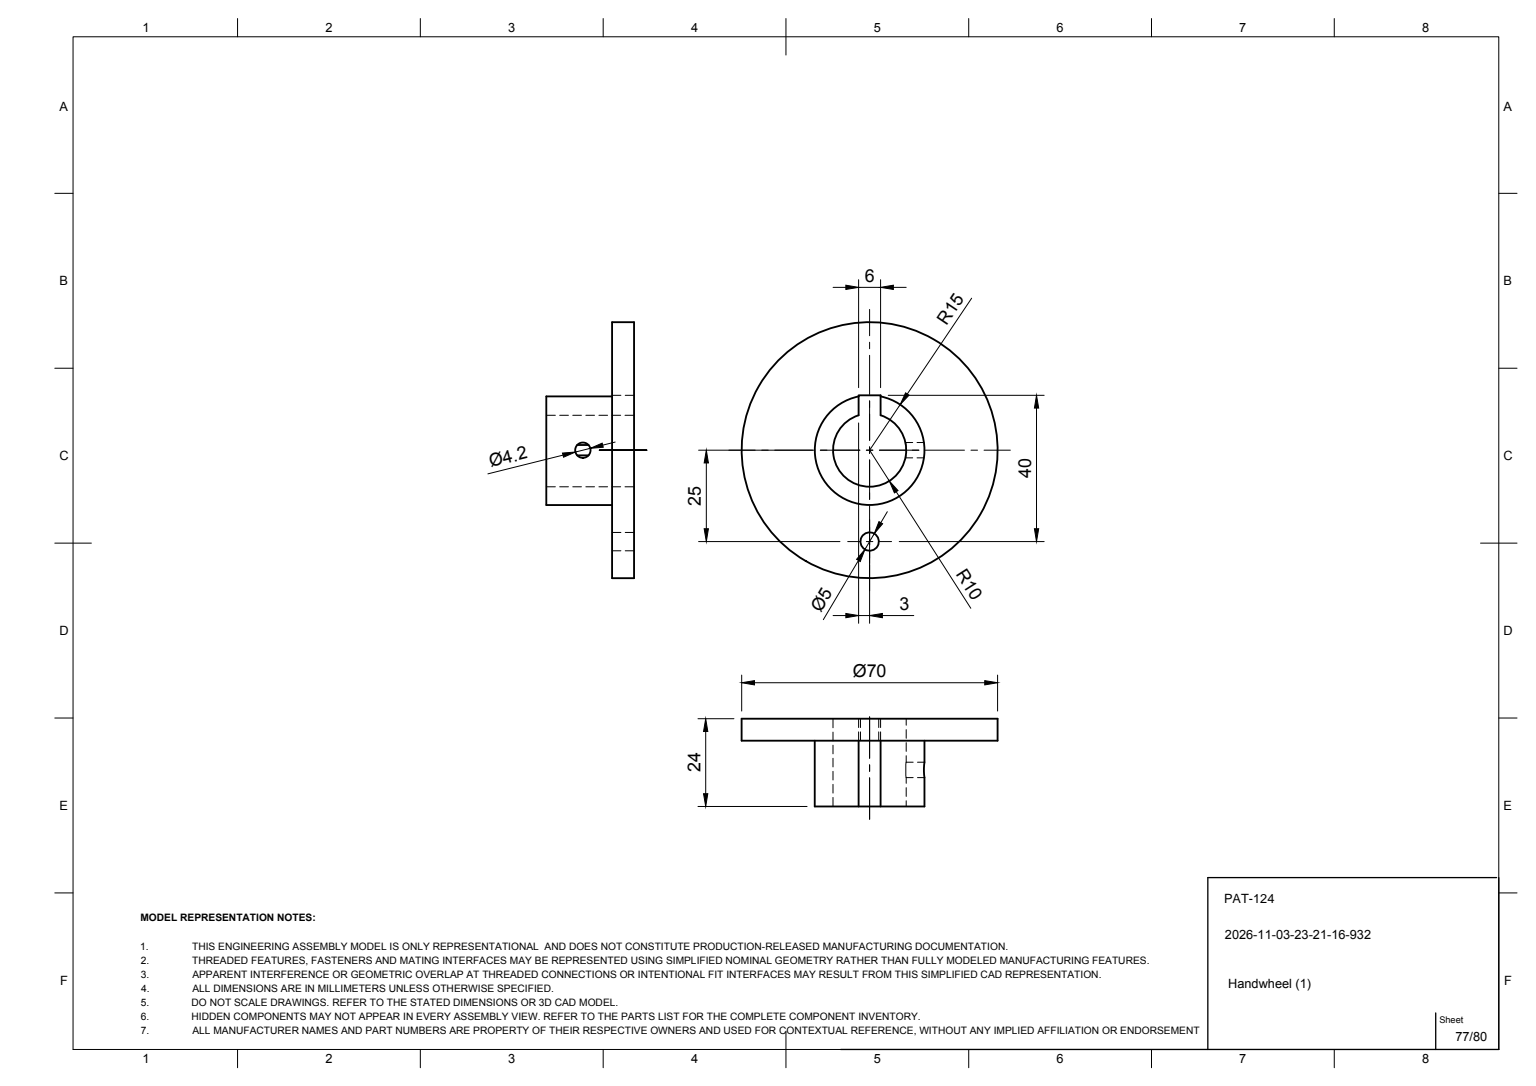
ISO-10303-21;
HEADER;
/* Generated by software containing ST-Developer
 * from STEP Tools, Inc. (www.steptools.com) 
 */

FILE_DESCRIPTION(
/* description */ ('XY cross-slide table'),
/* implementation_level */ '2;1');

FILE_NAME(
/* name */ 'Handwheel (1).step',
/* time_stamp */ '2026-10-28T03:22:46-07:00',
/* author */ (''),
/* organization */ (''),
/* preprocessor_version */ 'ST-DEVELOPER v20.2',
/* originating_system */ 'Autodesk Translation Framework v15.17.0.0',
/* authorisation */ '');

FILE_SCHEMA (('AUTOMOTIVE_DESIGN { 1 0 10303 214 3 1 1 }'));
ENDSEC;

DATA;
#10=MECHANICAL_DESIGN_GEOMETRIC_PRESENTATION_REPRESENTATION('',(#1776),#62984);
#1376=B_SPLINE_CURVE_WITH_KNOTS('',3,(#62407,#62408,#62409,#62410,#62411,
#62412),.UNSPECIFIED.,.F.,.F.,(4,2,4),(0.803821788694078,0.872950991853625,
0.952307212900975),.UNSPECIFIED.);
#1377=B_SPLINE_CURVE_WITH_KNOTS('',3,(#62415,#62416,#62417,#62418,#62419,
#62420,#62421,#62422,#62423,#62424),.UNSPECIFIED.,.F.,.F.,(4,2,2,2,4),(0.168950313426762,
0.238079516586309,0.317435737633658,0.396791958681008,0.465921161840561),
 .UNSPECIFIED.);
#1378=B_SPLINE_CURVE_WITH_KNOTS('',3,(#62425,#62426,#62427,#62428,#62429,
#62430),.UNSPECIFIED.,.F.,.F.,(4,2,4),(0.952307212900975,1.03166343394832,
1.10079263710787),.UNSPECIFIED.);
#1379=B_SPLINE_CURVE_WITH_KNOTS('',3,(#62434,#62435,#62436,#62437,#62438,
#62439,#62440,#62441,#62442,#62443),.UNSPECIFIED.,.F.,.F.,(4,2,2,2,4),(0.,
0.0792165807733642,0.158433161546728,0.237648697074572,0.316864232602417),
 .UNSPECIFIED.);
#1380=B_SPLINE_CURVE_WITH_KNOTS('',3,(#62444,#62445,#62446,#62447,#62448,
#62449,#62450,#62451,#62452,#62453,#62454,#62455,#62456,#62457,#62458,#62459,
#62460,#62461,#62462,#62463,#62464,#62465,#62466,#62467,#62468,#62469),
 .UNSPECIFIED.,.F.,.F.,(4,2,2,2,2,2,2,2,2,2,2,2,4),(0.316864232602417,0.396079768130261,
0.475295303658105,0.554511884431469,0.633728465204833,0.712945045978197,
0.792161626751562,0.871377162279406,0.95059269780725,1.02980823333509,1.10902376886294,
1.1882403496363,1.26745693040967),.UNSPECIFIED.);
#1580=SHAPE_REPRESENTATION_RELATIONSHIP('SRR','None',#63440,#1663);
#1663=ADVANCED_BREP_SHAPE_REPRESENTATION('',(#1881),#62977);
#1776=STYLED_ITEM('',(#63905),#1881);
#1881=MANIFOLD_SOLID_BREP('Body1',#23078);
#2282=FACE_BOUND('',#5836,.T.);
#2283=FACE_BOUND('',#5837,.T.);
#2284=FACE_BOUND('',#5839,.T.);
#2285=FACE_BOUND('',#5840,.T.);
#2286=FACE_BOUND('',#5843,.T.);
#2287=FACE_BOUND('',#5845,.T.);
#2825=PLANE('',#26309);
#2826=PLANE('',#26313);
#2827=PLANE('',#26314);
#2828=PLANE('',#26315);
#2829=PLANE('',#26316);
#2830=PLANE('',#26317);
#2831=PLANE('',#26320);
#2832=PLANE('',#26328);
#4119=FACE_OUTER_BOUND('',#5828,.T.);
#4120=FACE_OUTER_BOUND('',#5829,.T.);
#4121=FACE_OUTER_BOUND('',#5830,.T.);
#4122=FACE_OUTER_BOUND('',#5831,.T.);
#4123=FACE_OUTER_BOUND('',#5832,.T.);
#4124=FACE_OUTER_BOUND('',#5833,.T.);
#4125=FACE_OUTER_BOUND('',#5834,.T.);
#4126=FACE_OUTER_BOUND('',#5835,.T.);
#4127=FACE_OUTER_BOUND('',#5838,.T.);
#4128=FACE_OUTER_BOUND('',#5841,.T.);
#4129=FACE_OUTER_BOUND('',#5842,.T.);
#4130=FACE_OUTER_BOUND('',#5844,.T.);
#4131=FACE_OUTER_BOUND('',#5846,.T.);
#5828=EDGE_LOOP('',(#20774,#20775,#20776,#20777));
#5829=EDGE_LOOP('',(#20778,#20779));
#5830=EDGE_LOOP('',(#20780,#20781,#20782,#20783,#20784,#20785,#20786,#20787,
#20788));
#5831=EDGE_LOOP('',(#20789,#20790));
#5832=EDGE_LOOP('',(#20791,#20792,#20793,#20794,#20795,#20796));
#5833=EDGE_LOOP('',(#20797,#20798,#20799,#20800));
#5834=EDGE_LOOP('',(#20801,#20802,#20803,#20804,#20805,#20806));
#5835=EDGE_LOOP('',(#20807));
#5836=EDGE_LOOP('',(#20808));
#5837=EDGE_LOOP('',(#20809,#20810,#20811,#20812));
#5838=EDGE_LOOP('',(#20813));
#5839=EDGE_LOOP('',(#20814));
#5840=EDGE_LOOP('',(#20815,#20816,#20817,#20818));
#5841=EDGE_LOOP('',(#20819,#20820,#20821,#20822));
#5842=EDGE_LOOP('',(#20823,#20824,#20825,#20826));
#5843=EDGE_LOOP('',(#20827,#20828,#20829,#20830,#20831));
#5844=EDGE_LOOP('',(#20832,#20833,#20834,#20835));
#5845=EDGE_LOOP('',(#20836,#20837));
#5846=EDGE_LOOP('',(#20838,#20839,#20840,#20841));
#7299=LINE('',#62397,#8786);
#7300=LINE('',#62402,#8787);
#7301=LINE('',#62432,#8788);
#7302=LINE('',#62471,#8789);
#7303=LINE('',#62475,#8790);
#7304=LINE('',#62477,#8791);
#7305=LINE('',#62479,#8792);
#7306=LINE('',#62481,#8793);
#7307=LINE('',#62483,#8794);
#7308=LINE('',#62484,#8795);
#7309=LINE('',#62487,#8796);
#7310=LINE('',#62489,#8797);
#7311=LINE('',#62490,#8798);
#7312=LINE('',#62493,#8799);
#7313=LINE('',#62495,#8800);
#7314=LINE('',#62497,#8801);
#7315=LINE('',#62499,#8802);
#7316=LINE('',#62500,#8803);
#7317=LINE('',#62510,#8804);
#8786=VECTOR('',#32470,0.25);
#8787=VECTOR('',#32475,1.);
#8788=VECTOR('',#32482,0.210000000000001);
#8789=VECTOR('',#32485,1.);
#8790=VECTOR('',#32488,1.);
#8791=VECTOR('',#32489,1.);
#8792=VECTOR('',#32490,1.);
#8793=VECTOR('',#32491,1.);
#8794=VECTOR('',#32492,1.);
#8795=VECTOR('',#32493,1.);
#8796=VECTOR('',#32496,1.);
#8797=VECTOR('',#32497,1.);
#8798=VECTOR('',#32498,1.);
#8799=VECTOR('',#32501,1.);
#8800=VECTOR('',#32502,1.);
#8801=VECTOR('',#32503,1.);
#8802=VECTOR('',#32504,1.);
#8803=VECTOR('',#32505,1.);
#8804=VECTOR('',#32520,3.5);
#9739=CIRCLE('',#26307,0.25);
#9740=CIRCLE('',#26308,0.25);
#9741=CIRCLE('',#26310,0.210000000000001);
#9742=CIRCLE('',#26312,0.210000000000001);
#9743=CIRCLE('',#26318,3.5);
#9744=CIRCLE('',#26319,1.);
#9745=CIRCLE('',#26321,3.5);
#9746=CIRCLE('',#26322,1.5);
#9747=CIRCLE('',#26325,1.);
#9748=CIRCLE('',#26327,1.5);
#11749=VERTEX_POINT('',#62394);
#11750=VERTEX_POINT('',#62396);
#11751=VERTEX_POINT('',#62400);
#11752=VERTEX_POINT('',#62401);
#11753=VERTEX_POINT('',#62405);
#11754=VERTEX_POINT('',#62406);
#11755=VERTEX_POINT('',#62413);
#11756=VERTEX_POINT('',#62431);
#11757=VERTEX_POINT('',#62433);
#11758=VERTEX_POINT('',#62473);
#11759=VERTEX_POINT('',#62474);
#11760=VERTEX_POINT('',#62476);
#11761=VERTEX_POINT('',#62478);
#11762=VERTEX_POINT('',#62480);
#11763=VERTEX_POINT('',#62482);
#11764=VERTEX_POINT('',#62486);
#11765=VERTEX_POINT('',#62488);
#11766=VERTEX_POINT('',#62492);
#11767=VERTEX_POINT('',#62494);
#11768=VERTEX_POINT('',#62496);
#11769=VERTEX_POINT('',#62498);
#11770=VERTEX_POINT('',#62502);
#11771=VERTEX_POINT('',#62506);
#14771=EDGE_CURVE('',#11749,#11749,#9739,.T.);
#14772=EDGE_CURVE('',#11749,#11750,#7299,.T.);
#14773=EDGE_CURVE('',#11750,#11750,#9740,.T.);
#14774=EDGE_CURVE('',#11751,#11752,#7300,.T.);
#14775=EDGE_CURVE('',#11751,#11752,#9741,.T.);
#14776=EDGE_CURVE('',#11753,#11754,#1376,.T.);
#14777=EDGE_CURVE('',#11755,#11753,#9742,.T.);
#14778=EDGE_CURVE('',#11752,#11755,#1377,.T.);
#14779=EDGE_CURVE('',#11754,#11751,#1378,.T.);
#14780=EDGE_CURVE('',#11754,#11756,#7301,.T.);
#14781=EDGE_CURVE('',#11757,#11756,#1379,.T.);
#14782=EDGE_CURVE('',#11756,#11757,#1380,.T.);
#14783=EDGE_CURVE('',#11755,#11753,#7302,.T.);
#14784=EDGE_CURVE('',#11758,#11759,#7303,.T.);
#14785=EDGE_CURVE('',#11760,#11758,#7304,.T.);
#14786=EDGE_CURVE('',#11761,#11760,#7305,.T.);
#14787=EDGE_CURVE('',#11762,#11761,#7306,.T.);
#14788=EDGE_CURVE('',#11763,#11762,#7307,.T.);
#14789=EDGE_CURVE('',#11759,#11763,#7308,.T.);
#14790=EDGE_CURVE('',#11764,#11758,#7309,.T.);
#14791=EDGE_CURVE('',#11765,#11764,#7310,.T.);
#14792=EDGE_CURVE('',#11760,#11765,#7311,.T.);
#14793=EDGE_CURVE('',#11766,#11764,#7312,.T.);
#14794=EDGE_CURVE('',#11767,#11766,#7313,.T.);
#14795=EDGE_CURVE('',#11768,#11767,#7314,.T.);
#14796=EDGE_CURVE('',#11769,#11768,#7315,.T.);
#14797=EDGE_CURVE('',#11765,#11769,#7316,.T.);
#14798=EDGE_CURVE('',#11770,#11770,#9743,.T.);
#14799=EDGE_CURVE('',#11759,#11766,#9744,.T.);
#14800=EDGE_CURVE('',#11771,#11771,#9745,.T.);
#14801=EDGE_CURVE('',#11769,#11761,#9746,.T.);
#14802=EDGE_CURVE('',#11770,#11771,#7317,.T.);
#14803=EDGE_CURVE('',#11763,#11767,#9747,.T.);
#14804=EDGE_CURVE('',#11768,#11762,#9748,.T.);
#20774=ORIENTED_EDGE('',*,*,#14771,.F.);
#20775=ORIENTED_EDGE('',*,*,#14772,.T.);
#20776=ORIENTED_EDGE('',*,*,#14773,.F.);
#20777=ORIENTED_EDGE('',*,*,#14772,.F.);
#20778=ORIENTED_EDGE('',*,*,#14774,.F.);
#20779=ORIENTED_EDGE('',*,*,#14775,.T.);
#20780=ORIENTED_EDGE('',*,*,#14776,.F.);
#20781=ORIENTED_EDGE('',*,*,#14777,.F.);
#20782=ORIENTED_EDGE('',*,*,#14778,.F.);
#20783=ORIENTED_EDGE('',*,*,#14775,.F.);
#20784=ORIENTED_EDGE('',*,*,#14779,.F.);
#20785=ORIENTED_EDGE('',*,*,#14780,.T.);
#20786=ORIENTED_EDGE('',*,*,#14781,.F.);
#20787=ORIENTED_EDGE('',*,*,#14782,.F.);
#20788=ORIENTED_EDGE('',*,*,#14780,.F.);
#20789=ORIENTED_EDGE('',*,*,#14783,.F.);
#20790=ORIENTED_EDGE('',*,*,#14777,.T.);
#20791=ORIENTED_EDGE('',*,*,#14784,.F.);
#20792=ORIENTED_EDGE('',*,*,#14785,.F.);
#20793=ORIENTED_EDGE('',*,*,#14786,.F.);
#20794=ORIENTED_EDGE('',*,*,#14787,.F.);
#20795=ORIENTED_EDGE('',*,*,#14788,.F.);
#20796=ORIENTED_EDGE('',*,*,#14789,.F.);
#20797=ORIENTED_EDGE('',*,*,#14790,.F.);
#20798=ORIENTED_EDGE('',*,*,#14791,.F.);
#20799=ORIENTED_EDGE('',*,*,#14792,.F.);
#20800=ORIENTED_EDGE('',*,*,#14785,.T.);
#20801=ORIENTED_EDGE('',*,*,#14793,.F.);
#20802=ORIENTED_EDGE('',*,*,#14794,.F.);
#20803=ORIENTED_EDGE('',*,*,#14795,.F.);
#20804=ORIENTED_EDGE('',*,*,#14796,.F.);
#20805=ORIENTED_EDGE('',*,*,#14797,.F.);
#20806=ORIENTED_EDGE('',*,*,#14791,.T.);
#20807=ORIENTED_EDGE('',*,*,#14798,.T.);
#20808=ORIENTED_EDGE('',*,*,#14773,.T.);
#20809=ORIENTED_EDGE('',*,*,#14793,.T.);
#20810=ORIENTED_EDGE('',*,*,#14790,.T.);
#20811=ORIENTED_EDGE('',*,*,#14784,.T.);
#20812=ORIENTED_EDGE('',*,*,#14799,.T.);
#20813=ORIENTED_EDGE('',*,*,#14800,.F.);
#20814=ORIENTED_EDGE('',*,*,#14771,.T.);
#20815=ORIENTED_EDGE('',*,*,#14797,.T.);
#20816=ORIENTED_EDGE('',*,*,#14801,.T.);
#20817=ORIENTED_EDGE('',*,*,#14786,.T.);
#20818=ORIENTED_EDGE('',*,*,#14792,.T.);
#20819=ORIENTED_EDGE('',*,*,#14798,.F.);
#20820=ORIENTED_EDGE('',*,*,#14802,.T.);
#20821=ORIENTED_EDGE('',*,*,#14800,.T.);
#20822=ORIENTED_EDGE('',*,*,#14802,.F.);
#20823=ORIENTED_EDGE('',*,*,#14794,.T.);
#20824=ORIENTED_EDGE('',*,*,#14799,.F.);
#20825=ORIENTED_EDGE('',*,*,#14789,.T.);
#20826=ORIENTED_EDGE('',*,*,#14803,.T.);
#20827=ORIENTED_EDGE('',*,*,#14778,.T.);
#20828=ORIENTED_EDGE('',*,*,#14783,.T.);
#20829=ORIENTED_EDGE('',*,*,#14776,.T.);
#20830=ORIENTED_EDGE('',*,*,#14779,.T.);
#20831=ORIENTED_EDGE('',*,*,#14774,.T.);
#20832=ORIENTED_EDGE('',*,*,#14796,.T.);
#20833=ORIENTED_EDGE('',*,*,#14804,.T.);
#20834=ORIENTED_EDGE('',*,*,#14787,.T.);
#20835=ORIENTED_EDGE('',*,*,#14801,.F.);
#20836=ORIENTED_EDGE('',*,*,#14781,.T.);
#20837=ORIENTED_EDGE('',*,*,#14782,.T.);
#20838=ORIENTED_EDGE('',*,*,#14795,.T.);
#20839=ORIENTED_EDGE('',*,*,#14803,.F.);
#20840=ORIENTED_EDGE('',*,*,#14788,.T.);
#20841=ORIENTED_EDGE('',*,*,#14804,.F.);
#21636=CYLINDRICAL_SURFACE('',#26306,0.25);
#21637=CYLINDRICAL_SURFACE('',#26311,0.210000000000001);
#21638=CYLINDRICAL_SURFACE('',#26323,3.5);
#21639=CYLINDRICAL_SURFACE('',#26324,1.);
#21640=CYLINDRICAL_SURFACE('',#26326,1.5);
#22900=ADVANCED_FACE('',(#4119),#21636,.F.);
#22901=ADVANCED_FACE('',(#4120),#2825,.T.);
#22902=ADVANCED_FACE('',(#4121),#21637,.F.);
#22903=ADVANCED_FACE('',(#4122),#2826,.T.);
#22904=ADVANCED_FACE('',(#4123),#2827,.F.);
#22905=ADVANCED_FACE('',(#4124),#2828,.F.);
#22906=ADVANCED_FACE('',(#4125),#2829,.F.);
#22907=ADVANCED_FACE('',(#4126,#2282,#2283),#2830,.T.);
#22908=ADVANCED_FACE('',(#4127,#2284,#2285),#2831,.F.);
#22909=ADVANCED_FACE('',(#4128),#21638,.T.);
#22910=ADVANCED_FACE('',(#4129,#2286),#21639,.F.);
#22911=ADVANCED_FACE('',(#4130,#2287),#21640,.T.);
#22912=ADVANCED_FACE('',(#4131),#2832,.F.);
#23078=CLOSED_SHELL('',(#22900,#22901,#22902,#22903,#22904,#22905,#22906,
#22907,#22908,#22909,#22910,#22911,#22912));
#26305=AXIS2_PLACEMENT_3D('',#62392,#32464,#32465);
#26306=AXIS2_PLACEMENT_3D('',#62393,#32466,#32467);
#26307=AXIS2_PLACEMENT_3D('',#62395,#32468,#32469);
#26308=AXIS2_PLACEMENT_3D('',#62398,#32471,#32472);
#26309=AXIS2_PLACEMENT_3D('',#62399,#32473,#32474);
#26310=AXIS2_PLACEMENT_3D('',#62403,#32476,#32477);
#26311=AXIS2_PLACEMENT_3D('',#62404,#32478,#32479);
#26312=AXIS2_PLACEMENT_3D('',#62414,#32480,#32481);
#26313=AXIS2_PLACEMENT_3D('',#62470,#32483,#32484);
#26314=AXIS2_PLACEMENT_3D('',#62472,#32486,#32487);
#26315=AXIS2_PLACEMENT_3D('',#62485,#32494,#32495);
#26316=AXIS2_PLACEMENT_3D('',#62491,#32499,#32500);
#26317=AXIS2_PLACEMENT_3D('',#62501,#32506,#32507);
#26318=AXIS2_PLACEMENT_3D('',#62503,#32508,#32509);
#26319=AXIS2_PLACEMENT_3D('',#62504,#32510,#32511);
#26320=AXIS2_PLACEMENT_3D('',#62505,#32512,#32513);
#26321=AXIS2_PLACEMENT_3D('',#62507,#32514,#32515);
#26322=AXIS2_PLACEMENT_3D('',#62508,#32516,#32517);
#26323=AXIS2_PLACEMENT_3D('',#62509,#32518,#32519);
#26324=AXIS2_PLACEMENT_3D('',#62511,#32521,#32522);
#26325=AXIS2_PLACEMENT_3D('',#62512,#32523,#32524);
#26326=AXIS2_PLACEMENT_3D('',#62513,#32525,#32526);
#26327=AXIS2_PLACEMENT_3D('',#62514,#32527,#32528);
#26328=AXIS2_PLACEMENT_3D('',#62515,#32529,#32530);
#32464=DIRECTION('axis',(0.,0.,1.));
#32465=DIRECTION('refdir',(1.,0.,0.));
#32466=DIRECTION('center_axis',(1.,0.,0.));
#32467=DIRECTION('ref_axis',(0.,0.,-1.));
#32468=DIRECTION('center_axis',(1.,0.,0.));
#32469=DIRECTION('ref_axis',(0.,0.,-1.));
#32470=DIRECTION('',(1.,0.,0.));
#32471=DIRECTION('center_axis',(-1.,0.,0.));
#32472=DIRECTION('ref_axis',(0.,0.,-1.));
#32473=DIRECTION('center_axis',(0.,1.,0.));
#32474=DIRECTION('ref_axis',(1.,0.,0.));
#32475=DIRECTION('',(1.,0.,0.));
#32476=DIRECTION('center_axis',(0.,1.,0.));
#32477=DIRECTION('ref_axis',(1.,0.,0.));
#32478=DIRECTION('center_axis',(0.,1.,0.));
#32479=DIRECTION('ref_axis',(1.,0.,0.));
#32480=DIRECTION('center_axis',(0.,1.,0.));
#32481=DIRECTION('ref_axis',(1.,0.,0.));
#32482=DIRECTION('',(0.,1.,0.));
#32483=DIRECTION('center_axis',(0.,1.,0.));
#32484=DIRECTION('ref_axis',(1.,0.,0.));
#32485=DIRECTION('',(-1.,0.,0.));
#32486=DIRECTION('center_axis',(0.,-1.,0.));
#32487=DIRECTION('ref_axis',(0.,0.,-1.));
#32488=DIRECTION('',(0.,0.,1.));
#32489=DIRECTION('',(1.,0.,0.));
#32490=DIRECTION('',(0.,0.,-1.));
#32491=DIRECTION('',(1.,0.,0.));
#32492=DIRECTION('',(0.,0.,-1.));
#32493=DIRECTION('',(-1.,0.,0.));
#32494=DIRECTION('center_axis',(0.,0.,-1.));
#32495=DIRECTION('ref_axis',(0.,1.,0.));
#32496=DIRECTION('',(0.,-1.,0.));
#32497=DIRECTION('',(1.,0.,0.));
#32498=DIRECTION('',(0.,1.,0.));
#32499=DIRECTION('center_axis',(0.,1.,0.));
#32500=DIRECTION('ref_axis',(0.,0.,1.));
#32501=DIRECTION('',(0.,0.,-1.));
#32502=DIRECTION('',(1.,0.,0.));
#32503=DIRECTION('',(0.,0.,1.));
#32504=DIRECTION('',(-1.,0.,0.));
#32505=DIRECTION('',(0.,0.,1.));
#32506=DIRECTION('center_axis',(1.,0.,0.));
#32507=DIRECTION('ref_axis',(0.,0.,-1.));
#32508=DIRECTION('center_axis',(1.,0.,0.));
#32509=DIRECTION('ref_axis',(0.,0.,-1.));
#32510=DIRECTION('center_axis',(-1.,0.,0.));
#32511=DIRECTION('ref_axis',(0.,0.,-1.));
#32512=DIRECTION('center_axis',(1.,0.,0.));
#32513=DIRECTION('ref_axis',(0.,0.,-1.));
#32514=DIRECTION('center_axis',(1.,0.,0.));
#32515=DIRECTION('ref_axis',(0.,0.,-1.));
#32516=DIRECTION('center_axis',(1.,0.,0.));
#32517=DIRECTION('ref_axis',(0.,0.,-1.));
#32518=DIRECTION('center_axis',(1.,0.,0.));
#32519=DIRECTION('ref_axis',(0.,0.,-1.));
#32520=DIRECTION('',(-1.,0.,0.));
#32521=DIRECTION('center_axis',(1.,0.,0.));
#32522=DIRECTION('ref_axis',(0.,1.22464679914735E-16,1.));
#32523=DIRECTION('center_axis',(-1.,0.,0.));
#32524=DIRECTION('ref_axis',(0.,0.,-1.));
#32525=DIRECTION('center_axis',(1.,0.,0.));
#32526=DIRECTION('ref_axis',(0.,1.22464679914735E-16,1.));
#32527=DIRECTION('center_axis',(1.,0.,0.));
#32528=DIRECTION('ref_axis',(0.,0.,-1.));
#32529=DIRECTION('center_axis',(1.,0.,0.));
#32530=DIRECTION('ref_axis',(0.,0.,-1.));
#62392=CARTESIAN_POINT('',(0.,0.,0.));
#62393=CARTESIAN_POINT('Origin',(28.7,0.,6.5));
#62394=CARTESIAN_POINT('',(28.8,-3.06161699786838E-17,6.75));
#62395=CARTESIAN_POINT('Origin',(28.8,0.,6.5));
#62396=CARTESIAN_POINT('',(29.4,3.06161699786838E-17,6.75));
#62397=CARTESIAN_POINT('',(28.7,-3.06161699786838E-17,6.75));
#62398=CARTESIAN_POINT('Origin',(29.4,0.,6.5));
#62399=CARTESIAN_POINT('Origin',(28.,0.99,4.));
#62400=CARTESIAN_POINT('',(27.844436508139,0.99,4.14106735979666));
#62401=CARTESIAN_POINT('',(28.155563491861,0.99,4.14106735979666));
#62402=CARTESIAN_POINT('',(27.,0.99,4.14106735979666));
#62403=CARTESIAN_POINT('Origin',(28.,0.99,4.));
#62404=CARTESIAN_POINT('Origin',(28.,0.99,4.));
#62405=CARTESIAN_POINT('',(27.844436508139,0.99,3.85893264020334));
#62406=CARTESIAN_POINT('',(27.79,1.,4.));
#62407=CARTESIAN_POINT('Ctrl Pts',(27.844436508139,0.99,3.85893264020334));
#62408=CARTESIAN_POINT('Ctrl Pts',(27.8287948476368,0.992457849824465,3.87618164330178));
#62409=CARTESIAN_POINT('Ctrl Pts',(27.815375956669,0.994938193049464,3.8970013568903));
#62410=CARTESIAN_POINT('Ctrl Pts',(27.7953025362756,0.998844492372413,3.94538588560165));
#62411=CARTESIAN_POINT('Ctrl Pts',(27.79,1.,3.97354792631755));
#62412=CARTESIAN_POINT('Ctrl Pts',(27.79,1.,4.));
#62413=CARTESIAN_POINT('',(28.155563491861,0.99,3.85893264020334));
#62414=CARTESIAN_POINT('Origin',(28.,0.99,4.));
#62415=CARTESIAN_POINT('Ctrl Pts',(28.155563491861,0.99,4.14106735979666));
#62416=CARTESIAN_POINT('Ctrl Pts',(28.1712051523632,0.992457849824465,4.12381835669823));
#62417=CARTESIAN_POINT('Ctrl Pts',(28.184624043331,0.994938193049464,4.1029986431097));
#62418=CARTESIAN_POINT('Ctrl Pts',(28.2046974637244,0.998844492372413,4.05461411439835));
#62419=CARTESIAN_POINT('Ctrl Pts',(28.21,1.,4.02645207368245));
#62420=CARTESIAN_POINT('Ctrl Pts',(28.21,1.,3.97354792631755));
#62421=CARTESIAN_POINT('Ctrl Pts',(28.2046974637244,0.998844492372413,3.94538588560165));
#62422=CARTESIAN_POINT('Ctrl Pts',(28.184624043331,0.994938193049464,3.8970013568903));
#62423=CARTESIAN_POINT('Ctrl Pts',(28.1712051523632,0.992457849824465,3.87618164330178));
#62424=CARTESIAN_POINT('Ctrl Pts',(28.155563491861,0.99,3.85893264020334));
#62425=CARTESIAN_POINT('Ctrl Pts',(27.79,1.,4.));
#62426=CARTESIAN_POINT('Ctrl Pts',(27.79,1.,4.02645207368245));
#62427=CARTESIAN_POINT('Ctrl Pts',(27.7953025362756,0.998844492372413,4.05461411439835));
#62428=CARTESIAN_POINT('Ctrl Pts',(27.815375956669,0.994938193049464,4.1029986431097));
#62429=CARTESIAN_POINT('Ctrl Pts',(27.8287948476368,0.992457849824465,4.12381835669823));
#62430=CARTESIAN_POINT('Ctrl Pts',(27.844436508139,0.99,4.14106735979666));
#62431=CARTESIAN_POINT('',(27.79,1.5,4.));
#62432=CARTESIAN_POINT('',(27.79,0.99,4.));
#62433=CARTESIAN_POINT('',(28.,1.48522725533839,4.21));
#62434=CARTESIAN_POINT('Ctrl Pts',(28.,1.48522725533839,4.21));
#62435=CARTESIAN_POINT('Ctrl Pts',(27.9735944730755,1.48522725533839,4.21));
#62436=CARTESIAN_POINT('Ctrl Pts',(27.9454529259093,1.48600415954412,4.20471573726959));
#62437=CARTESIAN_POINT('Ctrl Pts',(27.8937237310949,1.48880073282317,4.18327376303633));
#62438=CARTESIAN_POINT('Ctrl Pts',(27.870133075872,1.49077897157582,4.16711792397039));
#62439=CARTESIAN_POINT('Ctrl Pts',(27.832882321789,1.49448481141327,4.12986716988737));
#62440=CARTESIAN_POINT('Ctrl Pts',(27.8167262899986,1.49645455657129,4.10627640830576));
#62441=CARTESIAN_POINT('Ctrl Pts',(27.7952841751738,1.49923165515646,4.0545468514059));
#62442=CARTESIAN_POINT('Ctrl Pts',(27.79,1.5,4.02640517850928));
#62443=CARTESIAN_POINT('Ctrl Pts',(27.79,1.5,4.));
#62444=CARTESIAN_POINT('Ctrl Pts',(27.79,1.5,4.));
#62445=CARTESIAN_POINT('Ctrl Pts',(27.79,1.5,3.97359482149072));
#62446=CARTESIAN_POINT('Ctrl Pts',(27.7952841751738,1.49923165515646,3.9454531485941));
#62447=CARTESIAN_POINT('Ctrl Pts',(27.8167262899986,1.49645455657129,3.89372359169424));
#62448=CARTESIAN_POINT('Ctrl Pts',(27.832882321789,1.49448481141327,3.87013283011263));
#62449=CARTESIAN_POINT('Ctrl Pts',(27.870133075872,1.49077897157582,3.83288207602961));
#62450=CARTESIAN_POINT('Ctrl Pts',(27.8937237310949,1.48880073282317,3.81672623696367));
#62451=CARTESIAN_POINT('Ctrl Pts',(27.9454529259093,1.48600415954412,3.7952842627304));
#62452=CARTESIAN_POINT('Ctrl Pts',(27.9735944730755,1.48522725533839,3.79));
#62453=CARTESIAN_POINT('Ctrl Pts',(28.0264055269245,1.48522725533839,3.79));
#62454=CARTESIAN_POINT('Ctrl Pts',(28.0545470740907,1.48600415954412,3.7952842627304));
#62455=CARTESIAN_POINT('Ctrl Pts',(28.1062762689051,1.48880073282317,3.81672623696367));
#62456=CARTESIAN_POINT('Ctrl Pts',(28.129866924128,1.49077897157582,3.83288207602961));
#62457=CARTESIAN_POINT('Ctrl Pts',(28.167117678211,1.49448481141327,3.87013283011263));
#62458=CARTESIAN_POINT('Ctrl Pts',(28.1832737100014,1.49645455657129,3.89372359169424));
#62459=CARTESIAN_POINT('Ctrl Pts',(28.2047158248262,1.49923165515646,3.9454531485941));
#62460=CARTESIAN_POINT('Ctrl Pts',(28.21,1.5,3.97359482149072));
#62461=CARTESIAN_POINT('Ctrl Pts',(28.21,1.5,4.02640517850928));
#62462=CARTESIAN_POINT('Ctrl Pts',(28.2047158248262,1.49923165515646,4.0545468514059));
#62463=CARTESIAN_POINT('Ctrl Pts',(28.1832737100014,1.49645455657129,4.10627640830576));
#62464=CARTESIAN_POINT('Ctrl Pts',(28.167117678211,1.49448481141327,4.12986716988737));
#62465=CARTESIAN_POINT('Ctrl Pts',(28.129866924128,1.49077897157582,4.16711792397039));
#62466=CARTESIAN_POINT('Ctrl Pts',(28.1062762689051,1.48880073282317,4.18327376303633));
#62467=CARTESIAN_POINT('Ctrl Pts',(28.0545470740907,1.48600415954412,4.2047157372696));
#62468=CARTESIAN_POINT('Ctrl Pts',(28.0264055269245,1.48522725533839,4.21));
#62469=CARTESIAN_POINT('Ctrl Pts',(28.,1.48522725533839,4.21));
#62470=CARTESIAN_POINT('Origin',(28.,0.99,4.));
#62471=CARTESIAN_POINT('',(27.,0.99,3.85893264020334));
#62472=CARTESIAN_POINT('Origin',(26.9,-0.3,4.));
#62473=CARTESIAN_POINT('',(29.4,-0.3,2.5));
#62474=CARTESIAN_POINT('',(29.4,-0.3,3.04606079858305));
#62475=CARTESIAN_POINT('',(29.4,-0.3,4.));
#62476=CARTESIAN_POINT('',(28.8,-0.3,2.5));
#62477=CARTESIAN_POINT('',(26.9,-0.3,2.5));
#62478=CARTESIAN_POINT('',(28.8,-0.3,2.53030615433009));
#62479=CARTESIAN_POINT('',(28.8,-0.3,4.));
#62480=CARTESIAN_POINT('',(27.,-0.3,2.53030615433009));
#62481=CARTESIAN_POINT('',(27.,-0.3,2.53030615433009));
#62482=CARTESIAN_POINT('',(27.,-0.3,3.04606079858305));
#62483=CARTESIAN_POINT('',(27.,-0.3,4.));
#62484=CARTESIAN_POINT('',(27.,-0.3,3.04606079858305));
#62485=CARTESIAN_POINT('Origin',(26.9,-0.3,2.5));
#62486=CARTESIAN_POINT('',(29.4,0.3,2.5));
#62487=CARTESIAN_POINT('',(29.4,-0.15,2.5));
#62488=CARTESIAN_POINT('',(28.8,0.3,2.5));
#62489=CARTESIAN_POINT('',(26.9,0.3,2.5));
#62490=CARTESIAN_POINT('',(28.8,-0.15,2.5));
#62491=CARTESIAN_POINT('Origin',(26.9,0.3,2.5));
#62492=CARTESIAN_POINT('',(29.4,0.3,3.04606079858305));
#62493=CARTESIAN_POINT('',(29.4,0.3,3.25));
#62494=CARTESIAN_POINT('',(27.,0.3,3.04606079858305));
#62495=CARTESIAN_POINT('',(27.,0.3,3.04606079858305));
#62496=CARTESIAN_POINT('',(27.,0.3,2.53030615433009));
#62497=CARTESIAN_POINT('',(27.,0.3,3.25));
#62498=CARTESIAN_POINT('',(28.8,0.3,2.53030615433009));
#62499=CARTESIAN_POINT('',(27.,0.3,2.53030615433009));
#62500=CARTESIAN_POINT('',(28.8,0.3,3.25));
#62501=CARTESIAN_POINT('Origin',(29.4,0.,4.));
#62502=CARTESIAN_POINT('',(29.4,-4.28626379701574E-16,7.5));
#62503=CARTESIAN_POINT('Origin',(29.4,0.,4.));
#62504=CARTESIAN_POINT('Origin',(29.4,0.,4.));
#62505=CARTESIAN_POINT('Origin',(28.8,0.,4.));
#62506=CARTESIAN_POINT('',(28.8,-4.28626379701574E-16,7.5));
#62507=CARTESIAN_POINT('Origin',(28.8,0.,4.));
#62508=CARTESIAN_POINT('Origin',(28.8,0.,4.));
#62509=CARTESIAN_POINT('Origin',(28.8,0.,4.));
#62510=CARTESIAN_POINT('',(28.8,-4.28626379701574E-16,7.5));
#62511=CARTESIAN_POINT('Origin',(27.,0.,4.));
#62512=CARTESIAN_POINT('Origin',(27.,0.,4.));
#62513=CARTESIAN_POINT('Origin',(27.,0.,4.));
#62514=CARTESIAN_POINT('Origin',(27.,0.,4.));
#62515=CARTESIAN_POINT('Origin',(27.,0.,4.));
#62878=UNCERTAINTY_MEASURE_WITH_UNIT(LENGTH_MEASURE(0.001),#62985,
'DISTANCE_ACCURACY_VALUE',
'Maximum model space distance between geometric entities at asserted c
onnectivities');
#62885=UNCERTAINTY_MEASURE_WITH_UNIT(LENGTH_MEASURE(0.001),#62985,
'DISTANCE_ACCURACY_VALUE',
'Maximum model space distance between geometric entities at asserted c
onnectivities');
#62977=(
GEOMETRIC_REPRESENTATION_CONTEXT(3)
GLOBAL_UNCERTAINTY_ASSIGNED_CONTEXT((#62878))
GLOBAL_UNIT_ASSIGNED_CONTEXT((#62985,#62987,#62988))
REPRESENTATION_CONTEXT('','3D')
);
#62984=(
GEOMETRIC_REPRESENTATION_CONTEXT(3)
GLOBAL_UNCERTAINTY_ASSIGNED_CONTEXT((#62885))
GLOBAL_UNIT_ASSIGNED_CONTEXT((#62985,#62987,#62988))
REPRESENTATION_CONTEXT('','3D')
);
#62985=(
LENGTH_UNIT()
NAMED_UNIT(*)
SI_UNIT(.CENTI.,.METRE.)
);
#62987=(
NAMED_UNIT(*)
PLANE_ANGLE_UNIT()
SI_UNIT($,.RADIAN.)
);
#62988=(
NAMED_UNIT(*)
SI_UNIT($,.STERADIAN.)
SOLID_ANGLE_UNIT()
);
#63080=SHAPE_DEFINITION_REPRESENTATION(#63291,#63440);
#63291=PRODUCT_DEFINITION_SHAPE('',$,#63539);
#63440=SHAPE_REPRESENTATION('',(#26305),#62977);
#63447=PRODUCT_DEFINITION_CONTEXT('part definition',#63743,'design');
#63539=PRODUCT_DEFINITION('Handwheel (1)','Handwheel (1)',#63637,#63447);
#63637=PRODUCT_DEFINITION_FORMATION('',$,#63836);
#63743=APPLICATION_CONTEXT(
'Core Data for Automotive Mechanical Design Process');
#63744=PRODUCT_CONTEXT('part definition',#63743,'mechanical');
#63836=PRODUCT('Handwheel (1)','Handwheel (1)','Handwheel (1)',(#63744));
#63899=COLOUR_RGB('Sky Blue',0.24,0.69,0.87);
#63900=FILL_AREA_STYLE_COLOUR('',#63899);
#63901=FILL_AREA_STYLE('',(#63900));
#63902=SURFACE_STYLE_FILL_AREA(#63901);
#63903=SURFACE_SIDE_STYLE('',(#63902));
#63904=SURFACE_STYLE_USAGE(.BOTH.,#63903);
#63905=PRESENTATION_STYLE_ASSIGNMENT((#63904));
ENDSEC;
END-ISO-10303-21;
